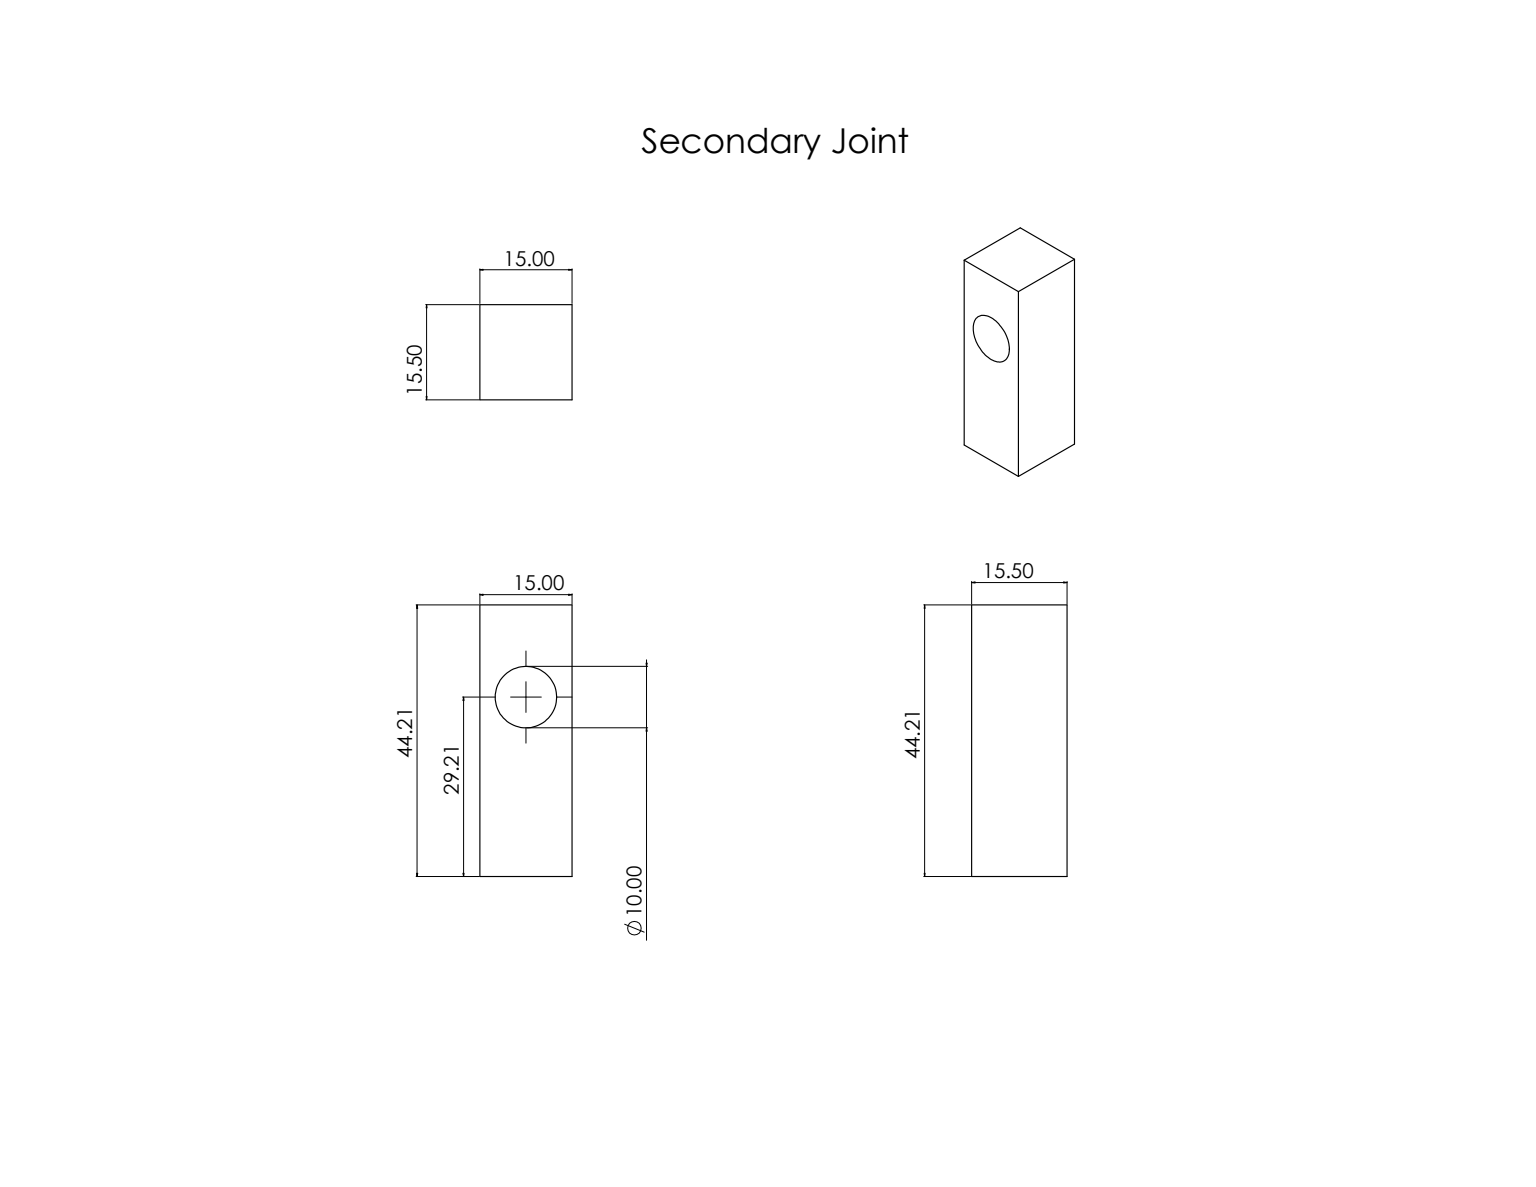
ISO-10303-21;
HEADER;
FILE_DESCRIPTION (('STEP AP214'),
    '1' );
FILE_NAME ('Secondary Joint.step',
    '2026-10-20T14:49:59',
    ( '' ),
    ( '' ),
    'SwSTEP 2.0',
    'SolidWorks 2025',
    '' );
FILE_SCHEMA (( 'AUTOMOTIVE_DESIGN' ));
ENDSEC;

DATA;
#53=( NAMED_UNIT ( * ) SI_UNIT ( $, .STERADIAN. ) SOLID_ANGLE_UNIT ( ) );
#100=LINE ( 'NONE', #5018, #2677 ) ;
#186=CARTESIAN_POINT ( 'NONE',  ( -8.793506896408096907, 120.5289575273812233, 54.43095569077609497 ) ) ;
#187=PLANE ( 'NONE',  #9912 ) ;
#191=AXIS2_PLACEMENT_3D ( 'NONE', #9432, #5392, #4342 ) ;
#198=AXIS2_PLACEMENT_3D ( 'NONE', #3567, #10035, #1182 ) ;
#229=ORIENTED_EDGE ( 'NONE', *, *, #1078, .F. ) ;
#263=VECTOR ( 'NONE', #2110, 1000.000000000000000 ) ;
#274=EDGE_CURVE ( 'NONE', #9380, #1455, #6041, .T. ) ;
#294=FACE_OUTER_BOUND ( 'NONE', #1619, .T. ) ;
#300=EDGE_CURVE ( 'NONE', #1692, #6075, #1817, .T. ) ;
#354=EDGE_CURVE ( 'NONE', #6075, #9366, #9784, .T. ) ;
#365=CIRCLE ( 'NONE', #1375, 5.000000000000007994 ) ;
#368=FACE_OUTER_BOUND ( 'NONE', #3797, .T. ) ;
#378=DIRECTION ( 'NONE',  ( 1.137729606058012035E-16, 0.000000000000000000, 1.000000000000000000 ) ) ;
#390=DIRECTION ( 'NONE',  ( -0.000000000000000000, -0.000000000000000000, -1.000000000000000000 ) ) ;
#396=DIRECTION ( 'NONE',  ( 9.101836848464095537E-17, 0.000000000000000000, 1.000000000000000000 ) ) ;
#399=VECTOR ( 'NONE', #9659, 1000.000000000000000 ) ;
#401=EDGE_CURVE ( 'NONE', #2275, #493, #4466, .T. ) ;
#431=ORIENTED_EDGE ( 'NONE', *, *, #8121, .T. ) ;
#455=CARTESIAN_POINT ( 'NONE',  ( -8.793506896408096907, 120.5289575273812233, 7.750000000000000000 ) ) ;
#466=ORIENTED_EDGE ( 'NONE', *, *, #354, .T. ) ;
#479=EDGE_LOOP ( 'NONE', ( #9318, #5776 ) ) ;
#491=VECTOR ( 'NONE', #5813, 1000.000000000000000 ) ;
#493=VERTEX_POINT ( 'NONE', #2817 ) ;
#525=EDGE_LOOP ( 'NONE', ( #1415, #3468, #7826, #6122 ) ) ;
#532=FACE_OUTER_BOUND ( 'NONE', #2911, .T. ) ;
#534=DIRECTION ( 'NONE',  ( -1.000000000000000000, 0.000000000000000000, 0.000000000000000000 ) ) ;
#606=VECTOR ( 'NONE', #7199, 1000.000000000000000 ) ;
#735=VERTEX_POINT ( 'NONE', #5031 ) ;
#797=ORIENTED_EDGE ( 'NONE', *, *, #9578, .T. ) ;
#845=ORIENTED_EDGE ( 'NONE', *, *, #1574, .T. ) ;
#884=EDGE_CURVE ( 'NONE', #2275, #9529, #6912, .T. ) ;
#914=PRODUCT_DEFINITION_CONTEXT ( 'detailed design', #6791, 'design' ) ;
#959=ORIENTED_EDGE ( 'NONE', *, *, #884, .F. ) ;
#1027=DIRECTION ( 'NONE',  ( 0.000000000000000000, 0.000000000000000000, -1.000000000000000000 ) ) ;
#1045=CARTESIAN_POINT ( 'NONE',  ( -8.793506896408100459, 76.32362273389503571, 54.43095569077609497 ) ) ;
#1078=EDGE_CURVE ( 'NONE', #9366, #5528, #100, .T. ) ;
#1153=VECTOR ( 'NONE', #8174, 1000.000000000000000 ) ;
#1164=EDGE_LOOP ( 'NONE', ( #3662, #4158, #8425, #4498 ) ) ;
#1182=DIRECTION ( 'NONE',  ( 1.000000000000000000, 0.000000000000000000, -1.734723475976804383E-16 ) ) ;
#1233=EDGE_CURVE ( 'NONE', #5528, #735, #9862, .T. ) ;
#1266=CARTESIAN_POINT ( 'NONE',  ( -16.29350689640809691, 105.5289575273812233, -7.750000000000000000 ) ) ;
#1309=ORIENTED_EDGE ( 'NONE', *, *, #6248, .F. ) ;
#1375=AXIS2_PLACEMENT_3D ( 'NONE', #1266, #7628, #6776 ) ;
#1415=ORIENTED_EDGE ( 'NONE', *, *, #7981, .F. ) ;
#1455=VERTEX_POINT ( 'NONE', #8622 ) ;
#1460=AXIS2_PLACEMENT_3D ( 'NONE', #7974, #8818, #5585 ) ;
#1462=CARTESIAN_POINT ( 'NONE',  ( -8.793506896408096907, 120.5289575273812233, -7.750000000000000000 ) ) ;
#1483=AXIS2_PLACEMENT_3D ( 'NONE', #3362, #5892, #1867 ) ;
#1574=EDGE_CURVE ( 'NONE', #1692, #8618, #4989, .T. ) ;
#1619=EDGE_LOOP ( 'NONE', ( #5586, #3361, #7908, #7176 ) ) ;
#1667=DIRECTION ( 'NONE',  ( 1.000000000000000000, 0.000000000000000000, -1.137729606058012035E-16 ) ) ;
#1688=( LENGTH_UNIT ( ) NAMED_UNIT ( * ) SI_UNIT ( .MILLI., .METRE. ) );
#1692=VERTEX_POINT ( 'NONE', #5416 ) ;
#1708=DIRECTION ( 'NONE',  ( -1.000000000000000000, 0.000000000000000000, 1.137729606058012035E-16 ) ) ;
#1729=CARTESIAN_POINT ( 'NONE',  ( -8.793506896408096907, 120.5289575273812233, -7.750000000000000000 ) ) ;
#1737=ORIENTED_EDGE ( 'NONE', *, *, #354, .F. ) ;
#1769=VECTOR ( 'NONE', #2995, 1000.000000000000000 ) ;
#1817=LINE ( 'NONE', #6590, #2828 ) ;
#1834=CARTESIAN_POINT ( 'NONE',  ( -23.79350689640809691, 120.5289575273812233, 54.43095569077609497 ) ) ;
#1867=DIRECTION ( 'NONE',  ( 0.000000000000000000, 0.000000000000000000, -1.000000000000000000 ) ) ;
#1872=CYLINDRICAL_SURFACE ( 'NONE', #10436, 4.729641367753004033 ) ;
#1899=AXIS2_PLACEMENT_3D ( 'NONE', #7238, #3907, #6336 ) ;
#1945=FACE_BOUND ( 'NONE', #479, .T. ) ;
#1957=AXIS2_PLACEMENT_3D ( 'NONE', #1834, #5062, #6496 ) ;
#1999=ORIENTED_EDGE ( 'NONE', *, *, #8846, .F. ) ;
#2013=CARTESIAN_POINT ( 'NONE',  ( -23.79350689640809691, 120.5289575273812233, 7.750000000000007105 ) ) ;
#2063=AXIS2_PLACEMENT_3D ( 'NONE', #186, #4990, #5102 ) ;
#2110=DIRECTION ( 'NONE',  ( -1.000000000000000000, 0.000000000000000000, 9.101836848464096770E-17 ) ) ;
#2114=ORIENTED_EDGE ( 'NONE', *, *, #6996, .F. ) ;
#2152=CYLINDRICAL_SURFACE ( 'NONE', #6213, 4.729641367753004033 ) ;
#2212=VERTEX_POINT ( 'NONE', #8302 ) ;
#2275=VERTEX_POINT ( 'NONE', #5124 ) ;
#2291=ORIENTED_EDGE ( 'NONE', *, *, #9502, .F. ) ;
#2300=CIRCLE ( 'NONE', #1460, 4.729641367753004033 ) ;
#2309=DIRECTION ( 'NONE',  ( -0.000000000000000000, -0.000000000000000000, -1.000000000000000000 ) ) ;
#2372=EDGE_LOOP ( 'NONE', ( #3117, #8725 ) ) ;
#2385=ADVANCED_FACE ( 'NONE', ( #2949 ), #2152, .F. ) ;
#2506=UNCERTAINTY_MEASURE_WITH_UNIT (LENGTH_MEASURE( 1.000000000000000082E-05 ), #6253, 'distance_accuracy_value', 'NONE');
#2512=FACE_OUTER_BOUND ( 'NONE', #1164, .T. ) ;
#2531=DIRECTION ( 'NONE',  ( 7.848480207562752404E-17, -1.000000000000000000, -7.143558635763577733E-33 ) ) ;
#2553=VERTEX_POINT ( 'NONE', #8082 ) ;
#2574=AXIS2_PLACEMENT_3D ( 'NONE', #6824, #8307, #3595 ) ;
#2647=CARTESIAN_POINT ( 'NONE',  ( -23.79350689640809691, 120.5289575273812233, -7.750000000000000000 ) ) ;
#2677=VECTOR ( 'NONE', #2531, 1000.000000000000000 ) ;
#2720=ORIENTED_EDGE ( 'NONE', *, *, #4427, .T. ) ;
#2736=VECTOR ( 'NONE', #3558, 1000.000000000000000 ) ;
#2749=ORIENTED_EDGE ( 'NONE', *, *, #1233, .F. ) ;
#2750=ADVANCED_FACE ( 'NONE', ( #9901 ), #3472, .F. ) ;
#2817=CARTESIAN_POINT ( 'NONE',  ( -21.29350689640810401, 105.5289575273812233, -7.749999999999999112 ) ) ;
#2828=VECTOR ( 'NONE', #1708, 1000.000000000000000 ) ;
#2911=EDGE_LOOP ( 'NONE', ( #1999, #431, #4347, #2114 ) ) ;
#2916=DIRECTION ( 'NONE',  ( 0.000000000000000000, -0.000000000000000000, 1.000000000000000000 ) ) ;
#2949=FACE_OUTER_BOUND ( 'NONE', #6460, .T. ) ;
#2960=CARTESIAN_POINT ( 'NONE',  ( -16.29350689640809691, 88.12362273389504708, -4.729641367753004033 ) ) ;
#2963=AXIS2_PLACEMENT_3D ( 'NONE', #3825, #3721, #534 ) ;
#2995=DIRECTION ( 'NONE',  ( 1.000000000000000000, 0.000000000000000000, -1.137729606058012035E-16 ) ) ;
#3117=ORIENTED_EDGE ( 'NONE', *, *, #6248, .T. ) ;
#3127=VECTOR ( 'NONE', #4690, 1000.000000000000000 ) ;
#3141=CARTESIAN_POINT ( 'NONE',  ( -23.79350689640809335, 76.32362273389503571, -7.750000000000000000 ) ) ;
#3159=EDGE_LOOP ( 'NONE', ( #8397, #7795, #2291, #6654 ) ) ;
#3161=MANIFOLD_SOLID_BREP ( 'Cut-Extrude10', #8758 ) ;
#3163=LINE ( 'NONE', #4748, #606 ) ;
#3228=ORIENTED_EDGE ( 'NONE', *, *, #8889, .F. ) ;
#3249=CIRCLE ( 'NONE', #1899, 4.729641367753004033 ) ;
#3305=CARTESIAN_POINT ( 'NONE',  ( 10.26554134690924691, 64.37996872128307757, 7.749999999999998224 ) ) ;
#3361=ORIENTED_EDGE ( 'NONE', *, *, #6996, .T. ) ;
#3362=CARTESIAN_POINT ( 'NONE',  ( -16.29350689640809691, 88.12362273389504708, 0.000000000000000000 ) ) ;
#3380=STYLED_ITEM('',(#10511),#3161);
#3389=CARTESIAN_POINT ( 'NONE',  ( -8.793506896408100459, 76.32362273389503571, 7.750000000000014211 ) ) ;
#3406=CIRCLE ( 'NONE', #198, 5.000000000000007994 ) ;
#3452=PRODUCT_DEFINITION_FORMATION_WITH_SPECIFIED_SOURCE ( 'ANY', '', #7892, .NOT_KNOWN. ) ;
#3468=ORIENTED_EDGE ( 'NONE', *, *, #10147, .T. ) ;
#3472=PLANE ( 'NONE',  #3890 ) ;
#3558=DIRECTION ( 'NONE',  ( 7.848480207562752404E-17, -1.000000000000000000, -8.929448294704472850E-33 ) ) ;
#3567=CARTESIAN_POINT ( 'NONE',  ( -16.29350689640809691, 105.5289575273812233, 7.750000000000000000 ) ) ;
#3595=DIRECTION ( 'NONE',  ( -1.000000000000000000, 0.000000000000000000, 9.101836848464095537E-17 ) ) ;
#3612=DIRECTION ( 'NONE',  ( 0.000000000000000000, 1.000000000000000000, 0.000000000000000000 ) ) ;
#3625=DIRECTION ( 'NONE',  ( -1.000000000000000000, 0.000000000000000000, 1.734723475976804383E-16 ) ) ;
#3627=EDGE_LOOP ( 'NONE', ( #9969, #845, #2720, #1737 ) ) ;
#3642=EDGE_CURVE ( 'NONE', #9384, #1692, #8503, .T. ) ;
#3662=ORIENTED_EDGE ( 'NONE', *, *, #300, .T. ) ;
#3695=CARTESIAN_POINT ( 'NONE',  ( -16.29350689640809691, 76.32362273389503571, 4.729641367753004033 ) ) ;
#3707=CARTESIAN_POINT ( 'NONE',  ( -23.79350689640809335, 120.5289575273812233, -7.750000000000000000 ) ) ;
#3721=DIRECTION ( 'NONE',  ( -0.000000000000000000, -0.000000000000000000, -1.000000000000000000 ) ) ;
#3744=ORIENTED_EDGE ( 'NONE', *, *, #10147, .F. ) ;
#3752=EDGE_LOOP ( 'NONE', ( #6562, #7468 ) ) ;
#3790=ADVANCED_FACE ( 'NONE', ( #10318 ), #5374, .F. ) ;
#3797=EDGE_LOOP ( 'NONE', ( #229, #7853, #3228, #2749 ) ) ;
#3825=CARTESIAN_POINT ( 'NONE',  ( -16.29350689640809691, 105.5289575273812233, 54.43095569077609497 ) ) ;
#3890=AXIS2_PLACEMENT_3D ( 'NONE', #4947, #5112, #8345 ) ;
#3898=MECHANICAL_DESIGN_GEOMETRIC_PRESENTATION_REPRESENTATION('',(#3380),#6255);
#3907=DIRECTION ( 'NONE',  ( 0.000000000000000000, -1.000000000000000000, 0.000000000000000000 ) ) ;
#3950=UNCERTAINTY_MEASURE_WITH_UNIT (LENGTH_MEASURE( 1.000000000000000082E-05 ), #1688, 'distance_accuracy_value', 'NONE');
#4117=FACE_OUTER_BOUND ( 'NONE', #5987, .T. ) ;
#4158=ORIENTED_EDGE ( 'NONE', *, *, #10407, .T. ) ;
#4224=VERTEX_POINT ( 'NONE', #5459 ) ;
#4231=CARTESIAN_POINT ( 'NONE',  ( -23.79350689640808980, 76.32362273389503571, -7.750000000000000000 ) ) ;
#4342=DIRECTION ( 'NONE',  ( 0.000000000000000000, 0.000000000000000000, -1.000000000000000000 ) ) ;
#4347=ORIENTED_EDGE ( 'NONE', *, *, #1233, .T. ) ;
#4427=EDGE_CURVE ( 'NONE', #8618, #9366, #9377, .T. ) ;
#4435=DIRECTION ( 'NONE',  ( 0.000000000000000000, 0.000000000000000000, -1.000000000000000000 ) ) ;
#4466=LINE ( 'NONE', #7754, #8936 ) ;
#4498=ORIENTED_EDGE ( 'NONE', *, *, #3642, .T. ) ;
#4601=AXIS2_PLACEMENT_3D ( 'NONE', #8586, #5983, #5928 ) ;
#4605=EDGE_CURVE ( 'NONE', #1455, #2553, #4797, .T. ) ;
#4637=LINE ( 'NONE', #1462, #3127 ) ;
#4668=EDGE_CURVE ( 'NONE', #9380, #9915, #3163, .T. ) ;
#4690=DIRECTION ( 'NONE',  ( 7.848480207562752404E-17, 1.000000000000000000, -7.143558635763577733E-33 ) ) ;
#4748=CARTESIAN_POINT ( 'NONE',  ( -16.29350689640809691, 88.12362273389504708, 4.729641367753004033 ) ) ;
#4756=ADVANCED_FACE ( 'NONE', ( #4117 ), #9096, .F. ) ;
#4797=LINE ( 'NONE', #2960, #6008 ) ;
#4836=AXIS2_PLACEMENT_3D ( 'NONE', #6056, #9947, #8393 ) ;
#4877=CARTESIAN_POINT ( 'NONE',  ( -16.29350689640809691, 105.5289575273812233, 54.43095569077609497 ) ) ;
#4937=VECTOR ( 'NONE', #9321, 1000.000000000000000 ) ;
#4944=EDGE_CURVE ( 'NONE', #2553, #9915, #2300, .T. ) ;
#4947=CARTESIAN_POINT ( 'NONE',  ( -23.79350689640809691, 120.5289575273812233, 54.43095569077609497 ) ) ;
#4989=LINE ( 'NONE', #9944, #5849 ) ;
#4990=DIRECTION ( 'NONE',  ( -1.000000000000000000, 7.848480207562752404E-17, 0.000000000000000000 ) ) ;
#4991=FACE_BOUND ( 'NONE', #5354, .T. ) ;
#5018=CARTESIAN_POINT ( 'NONE',  ( -23.79350689640809691, 120.5289575273812233, -7.750000000000000000 ) ) ;
#5031=CARTESIAN_POINT ( 'NONE',  ( -8.793506896408100459, 76.32362273389503571, -7.750000000000014211 ) ) ;
#5062=DIRECTION ( 'NONE',  ( 1.000000000000000000, 7.848480207562752404E-17, -0.000000000000000000 ) ) ;
#5101=DIRECTION ( 'NONE',  ( -0.000000000000000000, -0.000000000000000000, -1.000000000000000000 ) ) ;
#5102=DIRECTION ( 'NONE',  ( -7.848480207562752404E-17, -1.000000000000000000, 0.000000000000000000 ) ) ;
#5105=CARTESIAN_POINT ( 'NONE',  ( -16.29350689640809691, 88.12362273389504708, 0.000000000000000000 ) ) ;
#5112=DIRECTION ( 'NONE',  ( 0.000000000000000000, -1.000000000000000000, 0.000000000000000000 ) ) ;
#5124=CARTESIAN_POINT ( 'NONE',  ( -21.29350689640810401, 105.5289575273812233, 7.750000000000000888 ) ) ;
#5127=PLANE ( 'NONE',  #2574 ) ;
#5205=ADVANCED_FACE ( 'NONE', ( #6694 ), #1872, .F. ) ;
#5220=ADVANCED_FACE ( 'NONE', ( #8494 ), #6911, .T. ) ;
#5272=EDGE_CURVE ( 'NONE', #2212, #493, #5346, .T. ) ;
#5281=LINE ( 'NONE', #1045, #4937 ) ;
#5346=CIRCLE ( 'NONE', #7554, 5.000000000000007994 ) ;
#5354=EDGE_LOOP ( 'NONE', ( #959, #3744 ) ) ;
#5374=CYLINDRICAL_SURFACE ( 'NONE', #6553, 5.000000000000007994 ) ;
#5392=DIRECTION ( 'NONE',  ( 0.000000000000000000, -1.000000000000000000, 0.000000000000000000 ) ) ;
#5416=CARTESIAN_POINT ( 'NONE',  ( -8.793506896408096907, 120.5289575273812233, 7.750000000000020428 ) ) ;
#5459=CARTESIAN_POINT ( 'NONE',  ( -23.79350689640809335, 76.32362273389503571, 7.750000000000020428 ) ) ;
#5528=VERTEX_POINT ( 'NONE', #3141 ) ;
#5534=DIRECTION ( 'NONE',  ( -1.000000000000000000, 0.000000000000000000, 0.000000000000000000 ) ) ;
#5585=DIRECTION ( 'NONE',  ( 0.000000000000000000, 0.000000000000000000, -1.000000000000000000 ) ) ;
#5586=ORIENTED_EDGE ( 'NONE', *, *, #3642, .F. ) ;
#5625=ORIENTED_EDGE ( 'NONE', *, *, #274, .F. ) ;
#5676=ORIENTED_EDGE ( 'NONE', *, *, #4668, .T. ) ;
#5724=ORIENTED_EDGE ( 'NONE', *, *, #4944, .T. ) ;
#5747=SHAPE_REPRESENTATION ( 'Secondary Joint', ( #4601 ), #8362 ) ;
#5776=ORIENTED_EDGE ( 'NONE', *, *, #5272, .T. ) ;
#5813=DIRECTION ( 'NONE',  ( 1.000000000000000000, 0.000000000000000000, -9.101836848464096770E-17 ) ) ;
#5841=FACE_OUTER_BOUND ( 'NONE', #525, .T. ) ;
#5849=VECTOR ( 'NONE', #5101, 1000.000000000000000 ) ;
#5892=DIRECTION ( 'NONE',  ( 0.000000000000000000, -1.000000000000000000, 0.000000000000000000 ) ) ;
#5928=DIRECTION ( 'NONE',  ( 1.000000000000000000, 0.000000000000000000, 0.000000000000000000 ) ) ;
#5983=DIRECTION ( 'NONE',  ( 0.000000000000000000, 0.000000000000000000, 1.000000000000000000 ) ) ;
#5984=PLANE ( 'NONE',  #6652 ) ;
#5987=EDGE_LOOP ( 'NONE', ( #6477, #466, #8745, #9718 ) ) ;
#6008=VECTOR ( 'NONE', #6188, 1000.000000000000000 ) ;
#6014=CARTESIAN_POINT ( 'NONE',  ( -23.79350689640809691, 120.5289575273812233, 7.750000000000007105 ) ) ;
#6041=CIRCLE ( 'NONE', #1483, 4.729641367753004033 ) ;
#6056=CARTESIAN_POINT ( 'NONE',  ( -16.29350689640809691, 88.12362273389504708, 0.000000000000000000 ) ) ;
#6075=VERTEX_POINT ( 'NONE', #6014 ) ;
#6101=CIRCLE ( 'NONE', #191, 4.729641367753004033 ) ;
#6122=ORIENTED_EDGE ( 'NONE', *, *, #5272, .F. ) ;
#6188=DIRECTION ( 'NONE',  ( -0.000000000000000000, -1.000000000000000000, -0.000000000000000000 ) ) ;
#6213=AXIS2_PLACEMENT_3D ( 'NONE', #9260, #7775, #4435 ) ;
#6248=EDGE_CURVE ( 'NONE', #1455, #9380, #3249, .T. ) ;
#6253=( LENGTH_UNIT ( ) NAMED_UNIT ( * ) SI_UNIT ( .MILLI., .METRE. ) );
#6255=( GEOMETRIC_REPRESENTATION_CONTEXT ( 3 ) GLOBAL_UNCERTAINTY_ASSIGNED_CONTEXT ( ( #3950 ) ) GLOBAL_UNIT_ASSIGNED_CONTEXT ( ( #1688, #7307, #53 ) ) REPRESENTATION_CONTEXT ( 'NONE', 'WORKASPACE' ) );
#6336=DIRECTION ( 'NONE',  ( 0.000000000000000000, 0.000000000000000000, -1.000000000000000000 ) ) ;
#6337=SHAPE_DEFINITION_REPRESENTATION ( #8644, #5747 ) ;
#6460=EDGE_LOOP ( 'NONE', ( #9710, #1309, #7566, #5724 ) ) ;
#6477=ORIENTED_EDGE ( 'NONE', *, *, #10407, .F. ) ;
#6496=DIRECTION ( 'NONE',  ( -7.848480207562752404E-17, 1.000000000000000000, 0.000000000000000000 ) ) ;
#6553=AXIS2_PLACEMENT_3D ( 'NONE', #4877, #2309, #5534 ) ;
#6562=ORIENTED_EDGE ( 'NONE', *, *, #4944, .F. ) ;
#6590=CARTESIAN_POINT ( 'NONE',  ( -23.79350689640810401, 120.5289575273812233, 7.750000000000007105 ) ) ;
#6652=AXIS2_PLACEMENT_3D ( 'NONE', #9281, #3612, #2916 ) ;
#6654=ORIENTED_EDGE ( 'NONE', *, *, #401, .F. ) ;
#6694=FACE_OUTER_BOUND ( 'NONE', #7313, .T. ) ;
#6776=DIRECTION ( 'NONE',  ( -1.000000000000000000, 0.000000000000000000, 1.734723475976804383E-16 ) ) ;
#6780=CARTESIAN_POINT ( 'NONE',  ( -16.29350689640809691, 105.5289575273812233, 7.750000000000000000 ) ) ;
#6791=APPLICATION_CONTEXT ( 'automotive_design' ) ;
#6824=CARTESIAN_POINT ( 'NONE',  ( 10.26554134690924691, 64.37996872128307757, -7.750000000000000000 ) ) ;
#6911=PLANE ( 'NONE',  #4836 ) ;
#6912=CIRCLE ( 'NONE', #9631, 5.000000000000007994 ) ;
#6984=ADVANCED_FACE ( 'NONE', ( #368, #1945 ), #5127, .T. ) ;
#6996=EDGE_CURVE ( 'NONE', #9384, #735, #5281, .T. ) ;
#7073=VECTOR ( 'NONE', #9092, 1000.000000000000000 ) ;
#7134=LINE ( 'NONE', #9524, #1769 ) ;
#7176=ORIENTED_EDGE ( 'NONE', *, *, #1574, .F. ) ;
#7199=DIRECTION ( 'NONE',  ( -0.000000000000000000, -1.000000000000000000, -0.000000000000000000 ) ) ;
#7238=CARTESIAN_POINT ( 'NONE',  ( -16.29350689640809691, 88.12362273389504708, 0.000000000000000000 ) ) ;
#7277=ADVANCED_FACE ( 'NONE', ( #294 ), #7386, .F. ) ;
#7307=( NAMED_UNIT ( * ) PLANE_ANGLE_UNIT ( ) SI_UNIT ( $, .RADIAN. ) );
#7313=EDGE_LOOP ( 'NONE', ( #5625, #5676, #797, #9683 ) ) ;
#7386=PLANE ( 'NONE',  #2063 ) ;
#7416=DIRECTION ( 'NONE',  ( -0.000000000000000000, -0.000000000000000000, -1.000000000000000000 ) ) ;
#7468=ORIENTED_EDGE ( 'NONE', *, *, #9578, .F. ) ;
#7546=DIRECTION ( 'NONE',  ( -0.000000000000000000, -1.000000000000000000, -0.000000000000000000 ) ) ;
#7554=AXIS2_PLACEMENT_3D ( 'NONE', #9191, #396, #3625 ) ;
#7566=ORIENTED_EDGE ( 'NONE', *, *, #4605, .T. ) ;
#7628=DIRECTION ( 'NONE',  ( 9.101836848464095537E-17, 0.000000000000000000, 1.000000000000000000 ) ) ;
#7754=CARTESIAN_POINT ( 'NONE',  ( -21.29350689640810401, 105.5289575273812233, 54.43095569077609497 ) ) ;
#7775=DIRECTION ( 'NONE',  ( -0.000000000000000000, -1.000000000000000000, -0.000000000000000000 ) ) ;
#7795=ORIENTED_EDGE ( 'NONE', *, *, #7981, .T. ) ;
#7826=ORIENTED_EDGE ( 'NONE', *, *, #401, .T. ) ;
#7853=ORIENTED_EDGE ( 'NONE', *, *, #4427, .F. ) ;
#7892=PRODUCT ( 'Secondary Joint', 'Secondary Joint', '', ( #8617 ) ) ;
#7908=ORIENTED_EDGE ( 'NONE', *, *, #8889, .T. ) ;
#7941=ADVANCED_FACE ( 'NONE', ( #10183, #532 ), #5984, .F. ) ;
#7974=CARTESIAN_POINT ( 'NONE',  ( -16.29350689640809691, 76.32362273389503571, 0.000000000000000000 ) ) ;
#7981=EDGE_CURVE ( 'NONE', #9529, #2212, #8690, .T. ) ;
#8074=DIRECTION ( 'NONE',  ( 1.137729606058012035E-16, 0.000000000000000000, 1.000000000000000000 ) ) ;
#8082=CARTESIAN_POINT ( 'NONE',  ( -16.29350689640809691, 76.32362273389503571, -4.729641367753004033 ) ) ;
#8121=EDGE_CURVE ( 'NONE', #4224, #5528, #9812, .T. ) ;
#8174=DIRECTION ( 'NONE',  ( -0.000000000000000000, -0.000000000000000000, -1.000000000000000000 ) ) ;
#8197=PRODUCT_DEFINITION ( 'UNKNOWN', '', #3452, #914 ) ;
#8302=CARTESIAN_POINT ( 'NONE',  ( -11.29350689640808802, 105.5289575273812233, -7.750000000000000888 ) ) ;
#8307=DIRECTION ( 'NONE',  ( -9.101836848464095537E-17, 0.000000000000000000, -1.000000000000000000 ) ) ;
#8311=CARTESIAN_POINT ( 'NONE',  ( -16.29350689640809691, 88.12362273389504708, 4.729641367753004033 ) ) ;
#8345=DIRECTION ( 'NONE',  ( 0.000000000000000000, -0.000000000000000000, -1.000000000000000000 ) ) ;
#8362=( GEOMETRIC_REPRESENTATION_CONTEXT ( 3 ) GLOBAL_UNCERTAINTY_ASSIGNED_CONTEXT ( ( #2506 ) ) GLOBAL_UNIT_ASSIGNED_CONTEXT ( ( #6253, #9494, #9315 ) ) REPRESENTATION_CONTEXT ( 'NONE', 'WORKASPACE' ) );
#8393=DIRECTION ( 'NONE',  ( 0.000000000000000000, -0.000000000000000000, -1.000000000000000000 ) ) ;
#8397=ORIENTED_EDGE ( 'NONE', *, *, #884, .T. ) ;
#8410=SHAPE_REPRESENTATION_RELATIONSHIP ( 'NONE' , 'NONE' ,  #5747, #10381 ) ;
#8422=APPLICATION_CONTEXT ( 'automotive_design' ) ;
#8425=ORIENTED_EDGE ( 'NONE', *, *, #8846, .T. ) ;
#8494=FACE_OUTER_BOUND ( 'NONE', #2372, .T. ) ;
#8503=LINE ( 'NONE', #455, #7073 ) ;
#8586=CARTESIAN_POINT ( 'NONE',  ( 0.000000000000000000, 0.000000000000000000, 0.000000000000000000 ) ) ;
#8617=PRODUCT_CONTEXT ( 'NONE', #8422, 'mechanical' ) ;
#8618=VERTEX_POINT ( 'NONE', #1729 ) ;
#8622=CARTESIAN_POINT ( 'NONE',  ( -16.29350689640809691, 88.12362273389504708, -4.729641367753004033 ) ) ;
#8644=PRODUCT_DEFINITION_SHAPE ( 'NONE', 'NONE',  #8197 ) ;
#8690=LINE ( 'NONE', #10391, #399 ) ;
#8725=ORIENTED_EDGE ( 'NONE', *, *, #274, .T. ) ;
#8745=ORIENTED_EDGE ( 'NONE', *, *, #1078, .T. ) ;
#8758=CLOSED_SHELL ( 'NONE', ( #5205, #3790, #2750, #7277, #7941, #4756, #9167, #8979, #6984, #2385, #5220 ) ) ;
#8818=DIRECTION ( 'NONE',  ( 0.000000000000000000, -1.000000000000000000, 0.000000000000000000 ) ) ;
#8846=EDGE_CURVE ( 'NONE', #4224, #9384, #7134, .T. ) ;
#8889=EDGE_CURVE ( 'NONE', #735, #8618, #4637, .T. ) ;
#8936=VECTOR ( 'NONE', #390, 1000.000000000000000 ) ;
#8979=ADVANCED_FACE ( 'NONE', ( #4991, #2512 ), #187, .T. ) ;
#9092=DIRECTION ( 'NONE',  ( 7.848480207562752404E-17, 1.000000000000000000, -8.929448294704472850E-33 ) ) ;
#9096=PLANE ( 'NONE',  #1957 ) ;
#9167=ADVANCED_FACE ( 'NONE', ( #5841 ), #9389, .F. ) ;
#9191=CARTESIAN_POINT ( 'NONE',  ( -16.29350689640809691, 105.5289575273812233, -7.750000000000000000 ) ) ;
#9260=CARTESIAN_POINT ( 'NONE',  ( -16.29350689640809691, 88.12362273389504708, 0.000000000000000000 ) ) ;
#9281=CARTESIAN_POINT ( 'NONE',  ( -23.79350689640809335, 76.32362273389503571, 54.43095569077609497 ) ) ;
#9315=( NAMED_UNIT ( * ) SI_UNIT ( $, .STERADIAN. ) SOLID_ANGLE_UNIT ( ) );
#9318=ORIENTED_EDGE ( 'NONE', *, *, #9502, .T. ) ;
#9321=DIRECTION ( 'NONE',  ( -0.000000000000000000, -0.000000000000000000, -1.000000000000000000 ) ) ;
#9332=DIRECTION ( 'NONE',  ( 1.000000000000000000, 0.000000000000000000, -1.734723475976804383E-16 ) ) ;
#9366=VERTEX_POINT ( 'NONE', #2647 ) ;
#9373=VECTOR ( 'NONE', #7416, 1000.000000000000000 ) ;
#9377=LINE ( 'NONE', #3707, #263 ) ;
#9380=VERTEX_POINT ( 'NONE', #8311 ) ;
#9384=VERTEX_POINT ( 'NONE', #3389 ) ;
#9389=CYLINDRICAL_SURFACE ( 'NONE', #2963, 5.000000000000007994 ) ;
#9432=CARTESIAN_POINT ( 'NONE',  ( -16.29350689640809691, 76.32362273389503571, 0.000000000000000000 ) ) ;
#9494=( NAMED_UNIT ( * ) PLANE_ANGLE_UNIT ( ) SI_UNIT ( $, .RADIAN. ) );
#9502=EDGE_CURVE ( 'NONE', #493, #2212, #365, .T. ) ;
#9524=CARTESIAN_POINT ( 'NONE',  ( -23.79350689640810046, 76.32362273389503571, 7.750000000000007105 ) ) ;
#9529=VERTEX_POINT ( 'NONE', #10174 ) ;
#9578=EDGE_CURVE ( 'NONE', #9915, #2553, #6101, .T. ) ;
#9631=AXIS2_PLACEMENT_3D ( 'NONE', #6780, #378, #9332 ) ;
#9659=DIRECTION ( 'NONE',  ( -0.000000000000000000, -0.000000000000000000, -1.000000000000000000 ) ) ;
#9683=ORIENTED_EDGE ( 'NONE', *, *, #4605, .F. ) ;
#9710=ORIENTED_EDGE ( 'NONE', *, *, #4668, .F. ) ;
#9718=ORIENTED_EDGE ( 'NONE', *, *, #8121, .F. ) ;
#9784=LINE ( 'NONE', #9835, #1153 ) ;
#9812=LINE ( 'NONE', #9918, #9373 ) ;
#9823=LINE ( 'NONE', #2013, #2736 ) ;
#9835=CARTESIAN_POINT ( 'NONE',  ( -23.79350689640809691, 120.5289575273812233, 54.43095569077609497 ) ) ;
#9862=LINE ( 'NONE', #4231, #491 ) ;
#9901=FACE_OUTER_BOUND ( 'NONE', #3627, .T. ) ;
#9912=AXIS2_PLACEMENT_3D ( 'NONE', #3305, #8074, #1667 ) ;
#9915=VERTEX_POINT ( 'NONE', #3695 ) ;
#9918=CARTESIAN_POINT ( 'NONE',  ( -23.79350689640809335, 76.32362273389503571, 54.43095569077609497 ) ) ;
#9944=CARTESIAN_POINT ( 'NONE',  ( -8.793506896408096907, 120.5289575273812233, 54.43095569077609497 ) ) ;
#9947=DIRECTION ( 'NONE',  ( 0.000000000000000000, -1.000000000000000000, 0.000000000000000000 ) ) ;
#9969=ORIENTED_EDGE ( 'NONE', *, *, #300, .F. ) ;
#10035=DIRECTION ( 'NONE',  ( 1.137729606058012035E-16, 0.000000000000000000, 1.000000000000000000 ) ) ;
#10147=EDGE_CURVE ( 'NONE', #9529, #2275, #3406, .T. ) ;
#10174=CARTESIAN_POINT ( 'NONE',  ( -11.29350689640808802, 105.5289575273812233, 7.749999999999999112 ) ) ;
#10183=FACE_BOUND ( 'NONE', #3752, .T. ) ;
#10318=FACE_OUTER_BOUND ( 'NONE', #3159, .T. ) ;
#10381=ADVANCED_BREP_SHAPE_REPRESENTATION ( '', ( #3161, #4601 ), #8362 ) ;
#10391=CARTESIAN_POINT ( 'NONE',  ( -11.29350689640808802, 105.5289575273812233, 54.43095569077609497 ) ) ;
#10407=EDGE_CURVE ( 'NONE', #6075, #4224, #9823, .T. ) ;
#10436=AXIS2_PLACEMENT_3D ( 'NONE', #5105, #7546, #1027 ) ;
#10505=COLOUR_RGB('Sky Blue',0.24,0.69,0.87);
#10506=FILL_AREA_STYLE_COLOUR('',#10505);
#10507=FILL_AREA_STYLE('',(#10506));
#10508=SURFACE_STYLE_FILL_AREA(#10507);
#10509=SURFACE_SIDE_STYLE('',(#10508));
#10510=SURFACE_STYLE_USAGE(.BOTH.,#10509);
#10511=PRESENTATION_STYLE_ASSIGNMENT((#10510));
ENDSEC;
END-ISO-10303-21;
